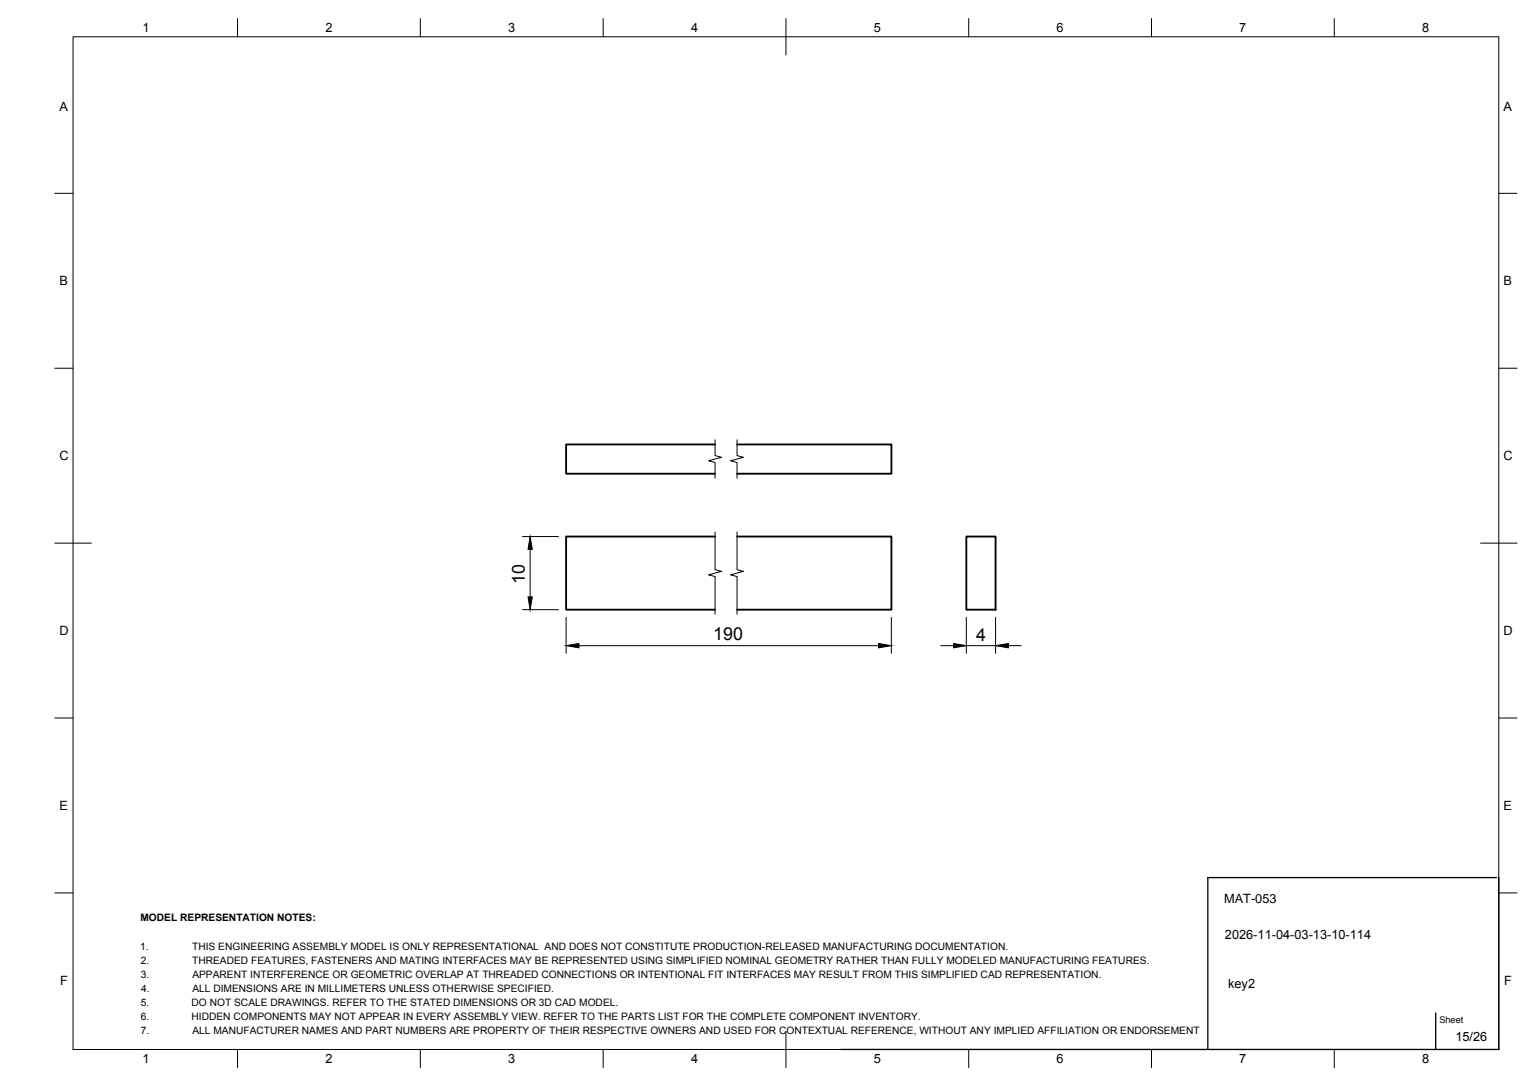
ISO-10303-21;
HEADER;
FILE_DESCRIPTION (('STEP AP214'),
    '1' );
FILE_NAME ('key2.step',
    '2026-10-10T03:43:58',
    ( '' ),
    ( '' ),
    'SwSTEP 2.0',
    'SolidWorks 2026',
    '' );
FILE_SCHEMA (( 'AUTOMOTIVE_DESIGN' ));
ENDSEC;

DATA;
#940=CARTESIAN_POINT ( 'NONE',  ( -20.00000000000002842, 3.680555555555560243, 4.000000000000000000 ) ) ;
#1677=AXIS2_PLACEMENT_3D ( 'NONE', #24509, #41705, #67758 ) ;
#2014=CARTESIAN_POINT ( 'NONE',  ( 169.9999999999999716, -6.319444444444440201, 4.000000000000000000 ) ) ;
#2159=ORIENTED_EDGE ( 'NONE', *, *, #27779, .F. ) ;
#2254=LINE ( 'NONE', #24051, #2264 ) ;
#2264=VECTOR ( 'NONE', #28628, 1000.000000000000000 ) ;
#2368=DIRECTION ( 'NONE',  ( -0.000000000000000000, 0.000000000000000000, 1.000000000000000000 ) ) ;
#2744=AXIS2_PLACEMENT_3D ( 'NONE', #62058, #62417, #30069 ) ;
#2822=VECTOR ( 'NONE', #54617, 1000.000000000000000 ) ;
#3358=EDGE_CURVE ( 'NONE', #60780, #10495, #49294, .T. ) ;
#3391=PRODUCT_CONTEXT ( 'NONE', #5772, 'mechanical' ) ;
#3506=EDGE_LOOP ( 'NONE', ( #56785, #7196, #50859, #10391 ) ) ;
#3533=DIRECTION ( 'NONE',  ( -0.000000000000000000, -0.000000000000000000, -1.000000000000000000 ) ) ;
#3545=VECTOR ( 'NONE', #38363, 1000.000000000000000 ) ;
#4584=AXIS2_PLACEMENT_3D ( 'NONE', #60998, #55723, #33927 ) ;
#5321=LINE ( 'NONE', #59115, #3545 ) ;
#5399=DIRECTION ( 'NONE',  ( 0.000000000000000000, -1.000000000000000000, 0.000000000000000000 ) ) ;
#5772=APPLICATION_CONTEXT ( 'automotive_design' ) ;
#6040=ADVANCED_FACE ( 'NONE', ( #29036 ), #51855, .T. ) ;
#6051=ORIENTED_EDGE ( 'NONE', *, *, #27779, .T. ) ;
#6429=EDGE_LOOP ( 'NONE', ( #43842, #33122, #54627, #18006 ) ) ;
#6747=DIRECTION ( 'NONE',  ( -0.000000000000000000, -0.000000000000000000, -1.000000000000000000 ) ) ;
#6941=PLANE ( 'NONE',  #35866 ) ;
#7196=ORIENTED_EDGE ( 'NONE', *, *, #3358, .F. ) ;
#7294=CARTESIAN_POINT ( 'NONE',  ( 0.000000000000000000, 0.000000000000000000, 0.000000000000000000 ) ) ;
#7905=SURFACE_STYLE_USAGE ( .BOTH. , #29353 ) ;
#8062=VECTOR ( 'NONE', #5399, 1000.000000000000000 ) ;
#8319=DIRECTION ( 'NONE',  ( 1.000000000000000000, 0.000000000000000000, 0.000000000000000000 ) ) ;
#8669=VERTEX_POINT ( 'NONE', #49098 ) ;
#8762=CARTESIAN_POINT ( 'NONE',  ( -20.00000000000002842, 3.680555555555560243, 4.000000000000000000 ) ) ;
#8828=CARTESIAN_POINT ( 'NONE',  ( 169.9999999999999716, 3.680555555555560243, 4.000000000000000000 ) ) ;
#9280=PRESENTATION_STYLE_ASSIGNMENT (( #7905 ) ) ;
#10050=DIRECTION ( 'NONE',  ( 0.000000000000000000, 0.000000000000000000, 1.000000000000000000 ) ) ;
#10080=EDGE_CURVE ( 'NONE', #29635, #60780, #19519, .T. ) ;
#10229=ORIENTED_EDGE ( 'NONE', *, *, #32472, .T. ) ;
#10292=ORIENTED_EDGE ( 'NONE', *, *, #10080, .T. ) ;
#10391=ORIENTED_EDGE ( 'NONE', *, *, #22790, .T. ) ;
#10495=VERTEX_POINT ( 'NONE', #57076 ) ;
#10788=DIRECTION ( 'NONE',  ( 1.000000000000000000, 0.000000000000000000, -0.000000000000000000 ) ) ;
#12441=ORIENTED_EDGE ( 'NONE', *, *, #3358, .T. ) ;
#12463=FACE_OUTER_BOUND ( 'NONE', #19621, .T. ) ;
#13504=UNCERTAINTY_MEASURE_WITH_UNIT (LENGTH_MEASURE( 1.000000000000000082E-05 ), #30058, 'distance_accuracy_value', 'NONE');
#13943=SHAPE_DEFINITION_REPRESENTATION ( #42230, #45625 ) ;
#14638=EDGE_CURVE ( 'NONE', #8669, #15703, #2254, .T. ) ;
#15036=AXIS2_PLACEMENT_3D ( 'NONE', #940, #10788, #42792 ) ;
#15332=PLANE ( 'NONE',  #55953 ) ;
#15418=VERTEX_POINT ( 'NONE', #36772 ) ;
#15546=LINE ( 'NONE', #38031, #21353 ) ;
#15703=VERTEX_POINT ( 'NONE', #33890 ) ;
#18006=ORIENTED_EDGE ( 'NONE', *, *, #44062, .F. ) ;
#18289=ORIENTED_EDGE ( 'NONE', *, *, #69173, .T. ) ;
#18383=CARTESIAN_POINT ( 'NONE',  ( -20.00000000000002842, -6.319444444444441089, 0.000000000000000000 ) ) ;
#19484=SURFACE_STYLE_FILL_AREA ( #32889 ) ;
#19519=LINE ( 'NONE', #68409, #23290 ) ;
#19621=EDGE_LOOP ( 'NONE', ( #31353, #25365, #69298, #12441 ) ) ;
#19715=LINE ( 'NONE', #8828, #55640 ) ;
#19771=EDGE_CURVE ( 'NONE', #64884, #10495, #31444, .T. ) ;
#20949=FACE_OUTER_BOUND ( 'NONE', #29473, .T. ) ;
#21353=VECTOR ( 'NONE', #47885, 1000.000000000000000 ) ;
#21743=VECTOR ( 'NONE', #61260, 1000.000000000000000 ) ;
#22423=FACE_OUTER_BOUND ( 'NONE', #6429, .T. ) ;
#22790=EDGE_CURVE ( 'NONE', #29635, #64884, #44373, .T. ) ;
#23290=VECTOR ( 'NONE', #40977, 1000.000000000000000 ) ;
#23734=FILL_AREA_STYLE_COLOUR ( '', #63970 ) ;
#24009=ADVANCED_FACE ( 'NONE', ( #31496 ), #63505, .F. ) ;
#24051=CARTESIAN_POINT ( 'NONE',  ( 169.9999999999999716, 3.680555555555560243, 4.000000000000000000 ) ) ;
#24239=CARTESIAN_POINT ( 'NONE',  ( 169.9999999999999716, 3.680555555555560243, 0.000000000000000000 ) ) ;
#24440=( NAMED_UNIT ( * ) SI_UNIT ( $, .STERADIAN. ) SOLID_ANGLE_UNIT ( ) );
#24509=CARTESIAN_POINT ( 'NONE',  ( -20.00000000000002842, 3.680555555555560243, 4.000000000000000000 ) ) ;
#25156=ORIENTED_EDGE ( 'NONE', *, *, #14638, .T. ) ;
#25365=ORIENTED_EDGE ( 'NONE', *, *, #60091, .F. ) ;
#25557=CARTESIAN_POINT ( 'NONE',  ( 169.9999999999999716, 3.680555555555560243, 4.000000000000000000 ) ) ;
#25976=CARTESIAN_POINT ( 'NONE',  ( 169.9999999999999716, 3.680555555555560243, 0.000000000000000000 ) ) ;
#26078=EDGE_LOOP ( 'NONE', ( #10229, #35989, #54763, #6051 ) ) ;
#26477=VECTOR ( 'NONE', #60734, 1000.000000000000000 ) ;
#27660=PLANE ( 'NONE',  #15036 ) ;
#27779=EDGE_CURVE ( 'NONE', #15703, #60845, #19715, .T. ) ;
#28628=DIRECTION ( 'NONE',  ( -0.000000000000000000, 1.000000000000000000, -0.000000000000000000 ) ) ;
#29036=FACE_OUTER_BOUND ( 'NONE', #46458, .T. ) ;
#29353=SURFACE_SIDE_STYLE ('',( #19484 ) ) ;
#29473=EDGE_LOOP ( 'NONE', ( #18289, #2159, #32314, #46701 ) ) ;
#29635=VERTEX_POINT ( 'NONE', #8762 ) ;
#30058=( LENGTH_UNIT ( ) NAMED_UNIT ( * ) SI_UNIT ( .MILLI., .METRE. ) );
#30069=DIRECTION ( 'NONE',  ( 1.000000000000000000, 0.000000000000000000, 0.000000000000000000 ) ) ;
#31075=UNCERTAINTY_MEASURE_WITH_UNIT (LENGTH_MEASURE( 1.000000000000000082E-05 ), #69381, 'distance_accuracy_value', 'NONE');
#31135=ADVANCED_FACE ( 'NONE', ( #20949 ), #15332, .F. ) ;
#31353=ORIENTED_EDGE ( 'NONE', *, *, #44062, .T. ) ;
#31444=LINE ( 'NONE', #32130, #8062 ) ;
#31496=FACE_OUTER_BOUND ( 'NONE', #26078, .T. ) ;
#31666=CLOSED_SHELL ( 'NONE', ( #68159, #36537, #31135, #24009, #6040, #64627 ) ) ;
#31750=SHAPE_REPRESENTATION_RELATIONSHIP ( 'NONE' , 'NONE' ,  #45625, #53289 ) ;
#32102=( NAMED_UNIT ( * ) PLANE_ANGLE_UNIT ( ) SI_UNIT ( $, .RADIAN. ) );
#32130=CARTESIAN_POINT ( 'NONE',  ( -20.00000000000002842, 3.680555555555560243, 0.000000000000000000 ) ) ;
#32314=ORIENTED_EDGE ( 'NONE', *, *, #14638, .F. ) ;
#32472=EDGE_CURVE ( 'NONE', #60845, #64884, #45189, .T. ) ;
#32790=( NAMED_UNIT ( * ) SI_UNIT ( $, .STERADIAN. ) SOLID_ANGLE_UNIT ( ) );
#32889=FILL_AREA_STYLE ('',( #23734 ) ) ;
#33122=ORIENTED_EDGE ( 'NONE', *, *, #32472, .F. ) ;
#33139=PRODUCT_DEFINITION_CONTEXT ( 'detailed design', #62394, 'design' ) ;
#33890=CARTESIAN_POINT ( 'NONE',  ( 169.9999999999999716, 3.680555555555560243, 4.000000000000000000 ) ) ;
#33927=DIRECTION ( 'NONE',  ( -1.000000000000000000, -4.565061778886334783E-18, 0.000000000000000000 ) ) ;
#34621=ORIENTED_EDGE ( 'NONE', *, *, #34802, .T. ) ;
#34802=EDGE_CURVE ( 'NONE', #60780, #8669, #15546, .T. ) ;
#34967=PLANE ( 'NONE',  #4584 ) ;
#35820=VECTOR ( 'NONE', #44844, 1000.000000000000000 ) ;
#35866=AXIS2_PLACEMENT_3D ( 'NONE', #7294, #2368, #43862 ) ;
#35918=( GEOMETRIC_REPRESENTATION_CONTEXT ( 3 ) GLOBAL_UNCERTAINTY_ASSIGNED_CONTEXT ( ( #13504 ) ) GLOBAL_UNIT_ASSIGNED_CONTEXT ( ( #30058, #36016, #24440 ) ) REPRESENTATION_CONTEXT ( 'NONE', 'WORKASPACE' ) );
#35989=ORIENTED_EDGE ( 'NONE', *, *, #22790, .F. ) ;
#36016=( NAMED_UNIT ( * ) PLANE_ANGLE_UNIT ( ) SI_UNIT ( $, .RADIAN. ) );
#36034=PRODUCT ( 'key2', 'key2', '', ( #3391 ) ) ;
#36537=ADVANCED_FACE ( 'NONE', ( #12463 ), #34967, .F. ) ;
#36772=CARTESIAN_POINT ( 'NONE',  ( 169.9999999999999716, -6.319444444444440201, 0.000000000000000000 ) ) ;
#37529=VECTOR ( 'NONE', #6747, 1000.000000000000000 ) ;
#37767=PRODUCT_DEFINITION_FORMATION_WITH_SPECIFIED_SOURCE ( 'ANY', '', #36034, .NOT_KNOWN. ) ;
#38031=CARTESIAN_POINT ( 'NONE',  ( -20.00000000000002842, -6.319444444444441089, 4.000000000000000000 ) ) ;
#38363=DIRECTION ( 'NONE',  ( -1.000000000000000000, -0.000000000000000000, -0.000000000000000000 ) ) ;
#39122=CARTESIAN_POINT ( 'NONE',  ( -20.00000000000002842, 3.680555555555560243, 4.000000000000000000 ) ) ;
#40977=DIRECTION ( 'NONE',  ( 0.000000000000000000, -1.000000000000000000, 0.000000000000000000 ) ) ;
#41705=DIRECTION ( 'NONE',  ( 0.000000000000000000, -1.000000000000000000, 0.000000000000000000 ) ) ;
#42143=CARTESIAN_POINT ( 'NONE',  ( -20.00000000000002842, -6.319444444444441089, 4.000000000000000000 ) ) ;
#42230=PRODUCT_DEFINITION_SHAPE ( 'NONE', 'NONE',  #58568 ) ;
#42792=DIRECTION ( 'NONE',  ( -0.000000000000000000, 0.000000000000000000, -1.000000000000000000 ) ) ;
#43842=ORIENTED_EDGE ( 'NONE', *, *, #19771, .F. ) ;
#43862=DIRECTION ( 'NONE',  ( 1.000000000000000000, 0.000000000000000000, 0.000000000000000000 ) ) ;
#44062=EDGE_CURVE ( 'NONE', #10495, #15418, #60601, .T. ) ;
#44373=LINE ( 'NONE', #39122, #21743 ) ;
#44558=DIRECTION ( 'NONE',  ( 0.000000000000000000, 0.000000000000000000, 1.000000000000000000 ) ) ;
#44844=DIRECTION ( 'NONE',  ( -1.000000000000000000, -0.000000000000000000, -0.000000000000000000 ) ) ;
#45189=LINE ( 'NONE', #66666, #35820 ) ;
#45625=SHAPE_REPRESENTATION ( 'key2', ( #66832 ), #63539 ) ;
#46458=EDGE_LOOP ( 'NONE', ( #10292, #34621, #25156, #68175 ) ) ;
#46612=VECTOR ( 'NONE', #50265, 1000.000000000000000 ) ;
#46701=ORIENTED_EDGE ( 'NONE', *, *, #60091, .T. ) ;
#46990=DIRECTION ( 'NONE',  ( -1.000000000000000000, 0.000000000000000000, 0.000000000000000000 ) ) ;
#47885=DIRECTION ( 'NONE',  ( 1.000000000000000000, 4.565061778886334783E-18, 0.000000000000000000 ) ) ;
#49047=CARTESIAN_POINT ( 'NONE',  ( -20.00000000000002842, 3.680555555555560243, 0.000000000000000000 ) ) ;
#49098=CARTESIAN_POINT ( 'NONE',  ( 169.9999999999999716, -6.319444444444440201, 4.000000000000000000 ) ) ;
#49294=LINE ( 'NONE', #66217, #37529 ) ;
#50265=DIRECTION ( 'NONE',  ( -0.000000000000000000, 1.000000000000000000, -0.000000000000000000 ) ) ;
#50530=CARTESIAN_POINT ( 'NONE',  ( 0.000000000000000000, 0.000000000000000000, 0.000000000000000000 ) ) ;
#50859=ORIENTED_EDGE ( 'NONE', *, *, #10080, .F. ) ;
#51474=EDGE_CURVE ( 'NONE', #15703, #29635, #5321, .T. ) ;
#51855=PLANE ( 'NONE',  #2744 ) ;
#53289=ADVANCED_BREP_SHAPE_REPRESENTATION ( '', ( #65002, #66832 ), #63539 ) ;
#54617=DIRECTION ( 'NONE',  ( 1.000000000000000000, 4.565061778886334783E-18, 0.000000000000000000 ) ) ;
#54627=ORIENTED_EDGE ( 'NONE', *, *, #69173, .F. ) ;
#54763=ORIENTED_EDGE ( 'NONE', *, *, #51474, .F. ) ;
#55640=VECTOR ( 'NONE', #3533, 1000.000000000000000 ) ;
#55723=DIRECTION ( 'NONE',  ( -4.565061778886334783E-18, 1.000000000000000000, 0.000000000000000000 ) ) ;
#55818=LINE ( 'NONE', #2014, #26477 ) ;
#55953=AXIS2_PLACEMENT_3D ( 'NONE', #25557, #46990, #10050 ) ;
#56785=ORIENTED_EDGE ( 'NONE', *, *, #19771, .T. ) ;
#57076=CARTESIAN_POINT ( 'NONE',  ( -20.00000000000002842, -6.319444444444441089, 0.000000000000000000 ) ) ;
#58568=PRODUCT_DEFINITION ( 'UNKNOWN', '', #37767, #33139 ) ;
#58974=FACE_OUTER_BOUND ( 'NONE', #3506, .T. ) ;
#59115=CARTESIAN_POINT ( 'NONE',  ( -20.00000000000002842, 3.680555555555560243, 4.000000000000000000 ) ) ;
#60091=EDGE_CURVE ( 'NONE', #8669, #15418, #55818, .T. ) ;
#60601=LINE ( 'NONE', #18383, #2822 ) ;
#60734=DIRECTION ( 'NONE',  ( -0.000000000000000000, -0.000000000000000000, -1.000000000000000000 ) ) ;
#60780=VERTEX_POINT ( 'NONE', #42143 ) ;
#60806=LINE ( 'NONE', #24239, #46612 ) ;
#60845=VERTEX_POINT ( 'NONE', #25976 ) ;
#60998=CARTESIAN_POINT ( 'NONE',  ( -20.00000000000002842, -6.319444444444441089, 4.000000000000000000 ) ) ;
#61260=DIRECTION ( 'NONE',  ( -0.000000000000000000, -0.000000000000000000, -1.000000000000000000 ) ) ;
#62058=CARTESIAN_POINT ( 'NONE',  ( 0.000000000000000000, 0.000000000000000000, 4.000000000000000000 ) ) ;
#62394=APPLICATION_CONTEXT ( 'automotive_design' ) ;
#62417=DIRECTION ( 'NONE',  ( -0.000000000000000000, 0.000000000000000000, 1.000000000000000000 ) ) ;
#63505=PLANE ( 'NONE',  #1677 ) ;
#63539=( GEOMETRIC_REPRESENTATION_CONTEXT ( 3 ) GLOBAL_UNCERTAINTY_ASSIGNED_CONTEXT ( ( #31075 ) ) GLOBAL_UNIT_ASSIGNED_CONTEXT ( ( #69381, #32102, #32790 ) ) REPRESENTATION_CONTEXT ( 'NONE', 'WORKASPACE' ) );
#63970=COLOUR_RGB ( '',0.7921568627450980005, 0.8196078431372548767, 0.9333333333333333481 ) ;
#64627=ADVANCED_FACE ( 'NONE', ( #22423 ), #6941, .F. ) ;
#64884=VERTEX_POINT ( 'NONE', #49047 ) ;
#65002=MANIFOLD_SOLID_BREP ( 'Boss-Extrude1', #31666 ) ;
#66217=CARTESIAN_POINT ( 'NONE',  ( -20.00000000000002842, -6.319444444444441089, 4.000000000000000000 ) ) ;
#66266=MECHANICAL_DESIGN_GEOMETRIC_PRESENTATION_REPRESENTATION('',(#68453),#35918);
#66666=CARTESIAN_POINT ( 'NONE',  ( -20.00000000000002842, 3.680555555555560243, 0.000000000000000000 ) ) ;
#66832=AXIS2_PLACEMENT_3D ( 'NONE', #50530, #44558, #8319 ) ;
#67758=DIRECTION ( 'NONE',  ( 0.000000000000000000, -0.000000000000000000, -1.000000000000000000 ) ) ;
#68159=ADVANCED_FACE ( 'NONE', ( #58974 ), #27660, .F. ) ;
#68175=ORIENTED_EDGE ( 'NONE', *, *, #51474, .T. ) ;
#68409=CARTESIAN_POINT ( 'NONE',  ( -20.00000000000002842, 3.680555555555560243, 4.000000000000000000 ) ) ;
#68453=STYLED_ITEM ( 'NONE', ( #9280 ), #65002 ) ;
#69173=EDGE_CURVE ( 'NONE', #15418, #60845, #60806, .T. ) ;
#69298=ORIENTED_EDGE ( 'NONE', *, *, #34802, .F. ) ;
#69381=( LENGTH_UNIT ( ) NAMED_UNIT ( * ) SI_UNIT ( .MILLI., .METRE. ) );
ENDSEC;
END-ISO-10303-21;
